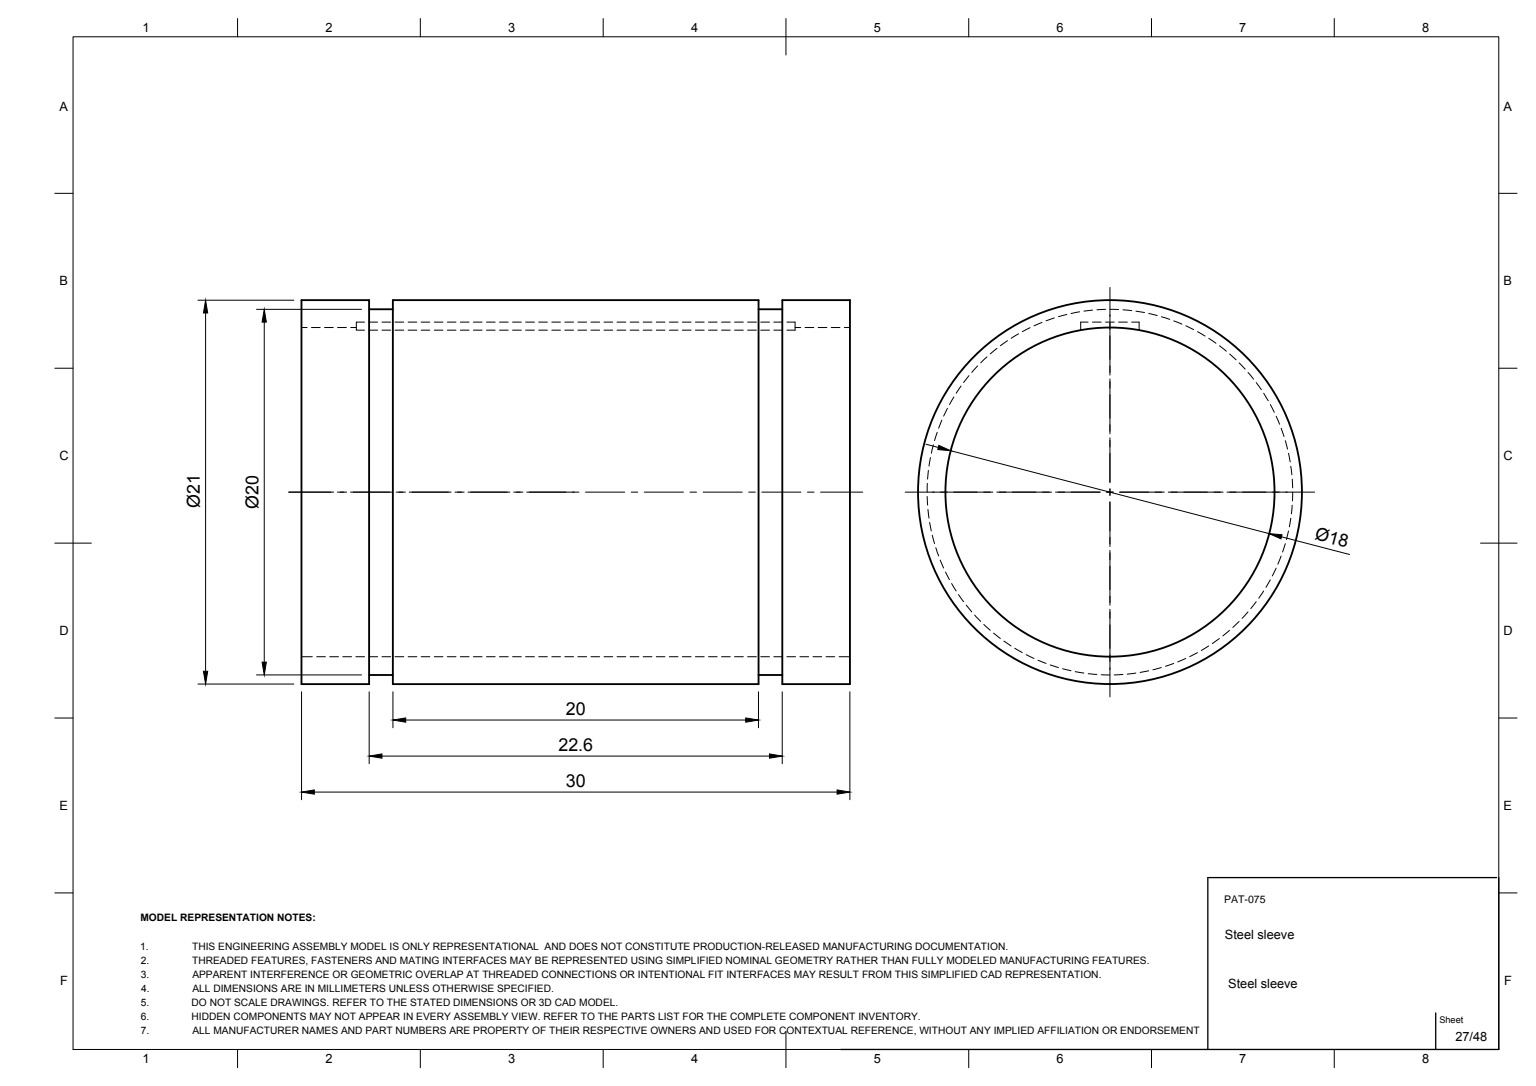
ISO-10303-21;
HEADER;
/* Generated by software containing ST-Developer
 * from STEP Tools, Inc. (www.steptools.com) 
 */

FILE_DESCRIPTION(
/* description */ ('Over-Centre Plunger Toggle Clamp on Slotted Fixture Frame'),
/* implementation_level */ '2;1');

FILE_NAME(
/* name */ 
'Steel sleeve.step',
/* time_stamp */ '2026-10-28T03:23:24-07:00',
/* author */ (''),
/* organization */ (''),
/* preprocessor_version */ 'ST-DEVELOPER v20.2',
/* originating_system */ 'Autodesk Translation Framework v15.17.0.0',
/* authorisation */ '');

FILE_SCHEMA (('AUTOMOTIVE_DESIGN { 1 0 10303 214 3 1 1 }'));
ENDSEC;

DATA;
#10=MECHANICAL_DESIGN_GEOMETRIC_PRESENTATION_REPRESENTATION('',(#542),#15212);
#450=SHAPE_REPRESENTATION_RELATIONSHIP('SRR','None',#15426,#492);
#492=ADVANCED_BREP_SHAPE_REPRESENTATION('',(#592),#15188);
#542=STYLED_ITEM('',(#15733),#592);
#592=MANIFOLD_SOLID_BREP('Body1',#8275);
#729=FACE_BOUND('',#1979,.T.);
#730=FACE_BOUND('',#1982,.T.);
#731=FACE_BOUND('',#1985,.T.);
#732=FACE_BOUND('',#1988,.T.);
#733=FACE_BOUND('',#1991,.T.);
#734=FACE_BOUND('',#1994,.T.);
#735=FACE_BOUND('',#1996,.T.);
#955=PLANE('',#9300);
#956=PLANE('',#9302);
#957=PLANE('',#9303);
#958=PLANE('',#9305);
#959=PLANE('',#9306);
#960=PLANE('',#9307);
#961=PLANE('',#9312);
#962=PLANE('',#9316);
#963=PLANE('',#9320);
#964=PLANE('',#9324);
#965=PLANE('',#9328);
#1369=FACE_OUTER_BOUND('',#1973,.T.);
#1370=FACE_OUTER_BOUND('',#1974,.T.);
#1371=FACE_OUTER_BOUND('',#1975,.T.);
#1372=FACE_OUTER_BOUND('',#1976,.T.);
#1373=FACE_OUTER_BOUND('',#1977,.T.);
#1374=FACE_OUTER_BOUND('',#1978,.T.);
#1375=FACE_OUTER_BOUND('',#1980,.T.);
#1376=FACE_OUTER_BOUND('',#1981,.T.);
#1377=FACE_OUTER_BOUND('',#1983,.T.);
#1378=FACE_OUTER_BOUND('',#1984,.T.);
#1379=FACE_OUTER_BOUND('',#1986,.T.);
#1380=FACE_OUTER_BOUND('',#1987,.T.);
#1381=FACE_OUTER_BOUND('',#1989,.T.);
#1382=FACE_OUTER_BOUND('',#1990,.T.);
#1383=FACE_OUTER_BOUND('',#1992,.T.);
#1384=FACE_OUTER_BOUND('',#1993,.T.);
#1385=FACE_OUTER_BOUND('',#1995,.T.);
#1973=EDGE_LOOP('',(#6841,#6842,#6843,#6844));
#1974=EDGE_LOOP('',(#6845,#6846,#6847,#6848));
#1975=EDGE_LOOP('',(#6849,#6850,#6851,#6852));
#1976=EDGE_LOOP('',(#6853,#6854,#6855,#6856));
#1977=EDGE_LOOP('',(#6857,#6858,#6859,#6860));
#1978=EDGE_LOOP('',(#6861));
#1979=EDGE_LOOP('',(#6862));
#1980=EDGE_LOOP('',(#6863,#6864,#6865,#6866));
#1981=EDGE_LOOP('',(#6867));
#1982=EDGE_LOOP('',(#6868));
#1983=EDGE_LOOP('',(#6869,#6870,#6871,#6872));
#1984=EDGE_LOOP('',(#6873));
#1985=EDGE_LOOP('',(#6874));
#1986=EDGE_LOOP('',(#6875,#6876,#6877,#6878));
#1987=EDGE_LOOP('',(#6879));
#1988=EDGE_LOOP('',(#6880));
#1989=EDGE_LOOP('',(#6881,#6882,#6883,#6884));
#1990=EDGE_LOOP('',(#6885));
#1991=EDGE_LOOP('',(#6886));
#1992=EDGE_LOOP('',(#6887,#6888,#6889,#6890));
#1993=EDGE_LOOP('',(#6891));
#1994=EDGE_LOOP('',(#6892));
#1995=EDGE_LOOP('',(#6893,#6894,#6895,#6896));
#1996=EDGE_LOOP('',(#6897,#6898,#6899,#6900));
#2625=LINE('',#14090,#3255);
#2626=LINE('',#14092,#3256);
#2627=LINE('',#14093,#3257);
#2628=LINE('',#14096,#3258);
#2629=LINE('',#14098,#3259);
#2630=LINE('',#14099,#3260);
#2631=LINE('',#14104,#3261);
#2632=LINE('',#14105,#3262);
#2633=LINE('',#14107,#3263);
#2634=LINE('',#14108,#3264);
#2635=LINE('',#14118,#3265);
#2636=LINE('',#14125,#3266);
#2637=LINE('',#14132,#3267);
#2638=LINE('',#14139,#3268);
#2639=LINE('',#14146,#3269);
#2640=LINE('',#14151,#3270);
#3255=VECTOR('',#11226,1.);
#3256=VECTOR('',#11227,1.);
#3257=VECTOR('',#11228,1.);
#3258=VECTOR('',#11231,1.);
#3259=VECTOR('',#11232,1.);
#3260=VECTOR('',#11233,1.);
#3261=VECTOR('',#11238,1.);
#3262=VECTOR('',#11239,1.);
#3263=VECTOR('',#11242,1.);
#3264=VECTOR('',#11243,1.);
#3265=VECTOR('',#11256,1.05);
#3266=VECTOR('',#11265,1.);
#3267=VECTOR('',#11274,1.05);
#3268=VECTOR('',#11283,1.);
#3269=VECTOR('',#11292,1.05);
#3270=VECTOR('',#11299,0.9);
#3713=CIRCLE('',#9301,0.9);
#3714=CIRCLE('',#9304,0.9);
#3715=CIRCLE('',#9308,1.05);
#3716=CIRCLE('',#9309,0.9);
#3717=CIRCLE('',#9311,1.05);
#3718=CIRCLE('',#9313,1.);
#3719=CIRCLE('',#9315,1.);
#3720=CIRCLE('',#9317,1.05);
#3721=CIRCLE('',#9319,1.05);
#3722=CIRCLE('',#9321,1.);
#3723=CIRCLE('',#9323,1.);
#3724=CIRCLE('',#9325,1.05);
#3725=CIRCLE('',#9327,1.05);
#3726=CIRCLE('',#9329,0.9);
#4291=VERTEX_POINT('',#14086);
#4292=VERTEX_POINT('',#14087);
#4293=VERTEX_POINT('',#14089);
#4294=VERTEX_POINT('',#14091);
#4295=VERTEX_POINT('',#14095);
#4296=VERTEX_POINT('',#14097);
#4297=VERTEX_POINT('',#14101);
#4298=VERTEX_POINT('',#14103);
#4299=VERTEX_POINT('',#14111);
#4300=VERTEX_POINT('',#14113);
#4301=VERTEX_POINT('',#14116);
#4302=VERTEX_POINT('',#14120);
#4303=VERTEX_POINT('',#14123);
#4304=VERTEX_POINT('',#14127);
#4305=VERTEX_POINT('',#14130);
#4306=VERTEX_POINT('',#14134);
#4307=VERTEX_POINT('',#14137);
#4308=VERTEX_POINT('',#14141);
#4309=VERTEX_POINT('',#14144);
#4310=VERTEX_POINT('',#14148);
#5181=EDGE_CURVE('',#4291,#4292,#3713,.T.);
#5182=EDGE_CURVE('',#4293,#4291,#2625,.T.);
#5183=EDGE_CURVE('',#4294,#4293,#2626,.T.);
#5184=EDGE_CURVE('',#4292,#4294,#2627,.T.);
#5185=EDGE_CURVE('',#4292,#4295,#2628,.T.);
#5186=EDGE_CURVE('',#4296,#4294,#2629,.T.);
#5187=EDGE_CURVE('',#4296,#4295,#2630,.T.);
#5188=EDGE_CURVE('',#4295,#4297,#3714,.T.);
#5189=EDGE_CURVE('',#4298,#4296,#2631,.T.);
#5190=EDGE_CURVE('',#4297,#4298,#2632,.T.);
#5191=EDGE_CURVE('',#4297,#4291,#2633,.T.);
#5192=EDGE_CURVE('',#4298,#4293,#2634,.T.);
#5193=EDGE_CURVE('',#4299,#4299,#3715,.T.);
#5194=EDGE_CURVE('',#4300,#4300,#3716,.T.);
#5195=EDGE_CURVE('',#4301,#4301,#3717,.T.);
#5196=EDGE_CURVE('',#4301,#4299,#2635,.T.);
#5197=EDGE_CURVE('',#4302,#4302,#3718,.T.);
#5198=EDGE_CURVE('',#4303,#4303,#3719,.T.);
#5199=EDGE_CURVE('',#4303,#4302,#2636,.T.);
#5200=EDGE_CURVE('',#4304,#4304,#3720,.T.);
#5201=EDGE_CURVE('',#4305,#4305,#3721,.T.);
#5202=EDGE_CURVE('',#4305,#4304,#2637,.T.);
#5203=EDGE_CURVE('',#4306,#4306,#3722,.T.);
#5204=EDGE_CURVE('',#4307,#4307,#3723,.T.);
#5205=EDGE_CURVE('',#4307,#4306,#2638,.T.);
#5206=EDGE_CURVE('',#4308,#4308,#3724,.T.);
#5207=EDGE_CURVE('',#4309,#4309,#3725,.T.);
#5208=EDGE_CURVE('',#4309,#4308,#2639,.T.);
#5209=EDGE_CURVE('',#4310,#4310,#3726,.T.);
#5210=EDGE_CURVE('',#4310,#4300,#2640,.T.);
#6841=ORIENTED_EDGE('',*,*,#5181,.F.);
#6842=ORIENTED_EDGE('',*,*,#5182,.F.);
#6843=ORIENTED_EDGE('',*,*,#5183,.F.);
#6844=ORIENTED_EDGE('',*,*,#5184,.F.);
#6845=ORIENTED_EDGE('',*,*,#5185,.F.);
#6846=ORIENTED_EDGE('',*,*,#5184,.T.);
#6847=ORIENTED_EDGE('',*,*,#5186,.F.);
#6848=ORIENTED_EDGE('',*,*,#5187,.T.);
#6849=ORIENTED_EDGE('',*,*,#5188,.F.);
#6850=ORIENTED_EDGE('',*,*,#5187,.F.);
#6851=ORIENTED_EDGE('',*,*,#5189,.F.);
#6852=ORIENTED_EDGE('',*,*,#5190,.F.);
#6853=ORIENTED_EDGE('',*,*,#5191,.F.);
#6854=ORIENTED_EDGE('',*,*,#5190,.T.);
#6855=ORIENTED_EDGE('',*,*,#5192,.T.);
#6856=ORIENTED_EDGE('',*,*,#5182,.T.);
#6857=ORIENTED_EDGE('',*,*,#5192,.F.);
#6858=ORIENTED_EDGE('',*,*,#5189,.T.);
#6859=ORIENTED_EDGE('',*,*,#5186,.T.);
#6860=ORIENTED_EDGE('',*,*,#5183,.T.);
#6861=ORIENTED_EDGE('',*,*,#5193,.F.);
#6862=ORIENTED_EDGE('',*,*,#5194,.T.);
#6863=ORIENTED_EDGE('',*,*,#5195,.F.);
#6864=ORIENTED_EDGE('',*,*,#5196,.T.);
#6865=ORIENTED_EDGE('',*,*,#5193,.T.);
#6866=ORIENTED_EDGE('',*,*,#5196,.F.);
#6867=ORIENTED_EDGE('',*,*,#5195,.T.);
#6868=ORIENTED_EDGE('',*,*,#5197,.F.);
#6869=ORIENTED_EDGE('',*,*,#5198,.F.);
#6870=ORIENTED_EDGE('',*,*,#5199,.T.);
#6871=ORIENTED_EDGE('',*,*,#5197,.T.);
#6872=ORIENTED_EDGE('',*,*,#5199,.F.);
#6873=ORIENTED_EDGE('',*,*,#5200,.F.);
#6874=ORIENTED_EDGE('',*,*,#5198,.T.);
#6875=ORIENTED_EDGE('',*,*,#5201,.F.);
#6876=ORIENTED_EDGE('',*,*,#5202,.T.);
#6877=ORIENTED_EDGE('',*,*,#5200,.T.);
#6878=ORIENTED_EDGE('',*,*,#5202,.F.);
#6879=ORIENTED_EDGE('',*,*,#5201,.T.);
#6880=ORIENTED_EDGE('',*,*,#5203,.F.);
#6881=ORIENTED_EDGE('',*,*,#5204,.F.);
#6882=ORIENTED_EDGE('',*,*,#5205,.T.);
#6883=ORIENTED_EDGE('',*,*,#5203,.T.);
#6884=ORIENTED_EDGE('',*,*,#5205,.F.);
#6885=ORIENTED_EDGE('',*,*,#5206,.F.);
#6886=ORIENTED_EDGE('',*,*,#5204,.T.);
#6887=ORIENTED_EDGE('',*,*,#5207,.F.);
#6888=ORIENTED_EDGE('',*,*,#5208,.T.);
#6889=ORIENTED_EDGE('',*,*,#5206,.T.);
#6890=ORIENTED_EDGE('',*,*,#5208,.F.);
#6891=ORIENTED_EDGE('',*,*,#5207,.T.);
#6892=ORIENTED_EDGE('',*,*,#5209,.F.);
#6893=ORIENTED_EDGE('',*,*,#5209,.T.);
#6894=ORIENTED_EDGE('',*,*,#5210,.T.);
#6895=ORIENTED_EDGE('',*,*,#5194,.F.);
#6896=ORIENTED_EDGE('',*,*,#5210,.F.);
#6897=ORIENTED_EDGE('',*,*,#5188,.T.);
#6898=ORIENTED_EDGE('',*,*,#5191,.T.);
#6899=ORIENTED_EDGE('',*,*,#5181,.T.);
#6900=ORIENTED_EDGE('',*,*,#5185,.T.);
#7701=CYLINDRICAL_SURFACE('',#9310,1.05);
#7702=CYLINDRICAL_SURFACE('',#9314,1.);
#7703=CYLINDRICAL_SURFACE('',#9318,1.05);
#7704=CYLINDRICAL_SURFACE('',#9322,1.);
#7705=CYLINDRICAL_SURFACE('',#9326,1.05);
#7706=CYLINDRICAL_SURFACE('',#9330,0.9);
#8041=ADVANCED_FACE('',(#1369),#955,.F.);
#8042=ADVANCED_FACE('',(#1370),#956,.F.);
#8043=ADVANCED_FACE('',(#1371),#957,.F.);
#8044=ADVANCED_FACE('',(#1372),#958,.F.);
#8045=ADVANCED_FACE('',(#1373),#959,.F.);
#8046=ADVANCED_FACE('',(#1374,#729),#960,.T.);
#8047=ADVANCED_FACE('',(#1375),#7701,.T.);
#8048=ADVANCED_FACE('',(#1376,#730),#961,.T.);
#8049=ADVANCED_FACE('',(#1377),#7702,.T.);
#8050=ADVANCED_FACE('',(#1378,#731),#962,.T.);
#8051=ADVANCED_FACE('',(#1379),#7703,.T.);
#8052=ADVANCED_FACE('',(#1380,#732),#963,.T.);
#8053=ADVANCED_FACE('',(#1381),#7704,.T.);
#8054=ADVANCED_FACE('',(#1382,#733),#964,.T.);
#8055=ADVANCED_FACE('',(#1383),#7705,.T.);
#8056=ADVANCED_FACE('',(#1384,#734),#965,.T.);
#8057=ADVANCED_FACE('',(#1385,#735),#7706,.F.);
#8275=CLOSED_SHELL('',(#8041,#8042,#8043,#8044,#8045,#8046,#8047,#8048,
#8049,#8050,#8051,#8052,#8053,#8054,#8055,#8056,#8057));
#9299=AXIS2_PLACEMENT_3D('',#14084,#11220,#11221);
#9300=AXIS2_PLACEMENT_3D('',#14085,#11222,#11223);
#9301=AXIS2_PLACEMENT_3D('',#14088,#11224,#11225);
#9302=AXIS2_PLACEMENT_3D('',#14094,#11229,#11230);
#9303=AXIS2_PLACEMENT_3D('',#14100,#11234,#11235);
#9304=AXIS2_PLACEMENT_3D('',#14102,#11236,#11237);
#9305=AXIS2_PLACEMENT_3D('',#14106,#11240,#11241);
#9306=AXIS2_PLACEMENT_3D('',#14109,#11244,#11245);
#9307=AXIS2_PLACEMENT_3D('',#14110,#11246,#11247);
#9308=AXIS2_PLACEMENT_3D('',#14112,#11248,#11249);
#9309=AXIS2_PLACEMENT_3D('',#14114,#11250,#11251);
#9310=AXIS2_PLACEMENT_3D('',#14115,#11252,#11253);
#9311=AXIS2_PLACEMENT_3D('',#14117,#11254,#11255);
#9312=AXIS2_PLACEMENT_3D('',#14119,#11257,#11258);
#9313=AXIS2_PLACEMENT_3D('',#14121,#11259,#11260);
#9314=AXIS2_PLACEMENT_3D('',#14122,#11261,#11262);
#9315=AXIS2_PLACEMENT_3D('',#14124,#11263,#11264);
#9316=AXIS2_PLACEMENT_3D('',#14126,#11266,#11267);
#9317=AXIS2_PLACEMENT_3D('',#14128,#11268,#11269);
#9318=AXIS2_PLACEMENT_3D('',#14129,#11270,#11271);
#9319=AXIS2_PLACEMENT_3D('',#14131,#11272,#11273);
#9320=AXIS2_PLACEMENT_3D('',#14133,#11275,#11276);
#9321=AXIS2_PLACEMENT_3D('',#14135,#11277,#11278);
#9322=AXIS2_PLACEMENT_3D('',#14136,#11279,#11280);
#9323=AXIS2_PLACEMENT_3D('',#14138,#11281,#11282);
#9324=AXIS2_PLACEMENT_3D('',#14140,#11284,#11285);
#9325=AXIS2_PLACEMENT_3D('',#14142,#11286,#11287);
#9326=AXIS2_PLACEMENT_3D('',#14143,#11288,#11289);
#9327=AXIS2_PLACEMENT_3D('',#14145,#11290,#11291);
#9328=AXIS2_PLACEMENT_3D('',#14147,#11293,#11294);
#9329=AXIS2_PLACEMENT_3D('',#14149,#11295,#11296);
#9330=AXIS2_PLACEMENT_3D('',#14150,#11297,#11298);
#11220=DIRECTION('axis',(0.,0.,1.));
#11221=DIRECTION('refdir',(1.,0.,0.));
#11222=DIRECTION('center_axis',(0.,1.,0.));
#11223=DIRECTION('ref_axis',(0.,0.,1.));
#11224=DIRECTION('center_axis',(0.,-1.,0.));
#11225=DIRECTION('ref_axis',(1.,0.,0.));
#11226=DIRECTION('',(-1.,0.,0.));
#11227=DIRECTION('',(0.,0.,-1.));
#11228=DIRECTION('',(1.,0.,0.));
#11229=DIRECTION('center_axis',(0.,0.,1.));
#11230=DIRECTION('ref_axis',(1.,0.,0.));
#11231=DIRECTION('',(0.,-1.,0.));
#11232=DIRECTION('',(0.,1.,0.));
#11233=DIRECTION('',(-1.,0.,0.));
#11234=DIRECTION('center_axis',(0.,-1.,0.));
#11235=DIRECTION('ref_axis',(0.,0.,-1.));
#11236=DIRECTION('center_axis',(0.,1.,0.));
#11237=DIRECTION('ref_axis',(1.,0.,0.));
#11238=DIRECTION('',(0.,0.,1.));
#11239=DIRECTION('',(1.,0.,0.));
#11240=DIRECTION('center_axis',(0.,0.,-1.));
#11241=DIRECTION('ref_axis',(-1.,0.,0.));
#11242=DIRECTION('',(0.,1.,0.));
#11243=DIRECTION('',(0.,1.,0.));
#11244=DIRECTION('center_axis',(1.,0.,0.));
#11245=DIRECTION('ref_axis',(0.,0.,-1.));
#11246=DIRECTION('center_axis',(0.,1.,0.));
#11247=DIRECTION('ref_axis',(0.,0.,1.));
#11248=DIRECTION('center_axis',(0.,-1.,0.));
#11249=DIRECTION('ref_axis',(1.,0.,0.));
#11250=DIRECTION('center_axis',(0.,-1.,0.));
#11251=DIRECTION('ref_axis',(1.,0.,0.));
#11252=DIRECTION('center_axis',(0.,-1.,0.));
#11253=DIRECTION('ref_axis',(1.,0.,0.));
#11254=DIRECTION('center_axis',(0.,-1.,0.));
#11255=DIRECTION('ref_axis',(1.,0.,0.));
#11256=DIRECTION('',(0.,1.,0.));
#11257=DIRECTION('center_axis',(0.,-1.,0.));
#11258=DIRECTION('ref_axis',(0.,0.,-1.));
#11259=DIRECTION('center_axis',(0.,-1.,0.));
#11260=DIRECTION('ref_axis',(1.,0.,0.));
#11261=DIRECTION('center_axis',(0.,-1.,0.));
#11262=DIRECTION('ref_axis',(1.,0.,0.));
#11263=DIRECTION('center_axis',(0.,-1.,0.));
#11264=DIRECTION('ref_axis',(1.,0.,0.));
#11265=DIRECTION('',(0.,1.,0.));
#11266=DIRECTION('center_axis',(0.,1.,0.));
#11267=DIRECTION('ref_axis',(0.,0.,1.));
#11268=DIRECTION('center_axis',(0.,-1.,0.));
#11269=DIRECTION('ref_axis',(1.,0.,0.));
#11270=DIRECTION('center_axis',(0.,-1.,0.));
#11271=DIRECTION('ref_axis',(1.,0.,0.));
#11272=DIRECTION('center_axis',(0.,-1.,0.));
#11273=DIRECTION('ref_axis',(1.,0.,0.));
#11274=DIRECTION('',(0.,1.,0.));
#11275=DIRECTION('center_axis',(0.,-1.,0.));
#11276=DIRECTION('ref_axis',(0.,0.,-1.));
#11277=DIRECTION('center_axis',(0.,-1.,0.));
#11278=DIRECTION('ref_axis',(1.,0.,0.));
#11279=DIRECTION('center_axis',(0.,-1.,0.));
#11280=DIRECTION('ref_axis',(1.,0.,0.));
#11281=DIRECTION('center_axis',(0.,-1.,0.));
#11282=DIRECTION('ref_axis',(1.,0.,0.));
#11283=DIRECTION('',(0.,1.,0.));
#11284=DIRECTION('center_axis',(0.,1.,0.));
#11285=DIRECTION('ref_axis',(0.,0.,1.));
#11286=DIRECTION('center_axis',(0.,-1.,0.));
#11287=DIRECTION('ref_axis',(1.,0.,0.));
#11288=DIRECTION('center_axis',(0.,-1.,0.));
#11289=DIRECTION('ref_axis',(1.,0.,0.));
#11290=DIRECTION('center_axis',(0.,-1.,0.));
#11291=DIRECTION('ref_axis',(1.,0.,0.));
#11292=DIRECTION('',(0.,1.,0.));
#11293=DIRECTION('center_axis',(0.,-1.,0.));
#11294=DIRECTION('ref_axis',(0.,0.,-1.));
#11295=DIRECTION('center_axis',(0.,-1.,0.));
#11296=DIRECTION('ref_axis',(1.,0.,0.));
#11297=DIRECTION('center_axis',(0.,-1.,0.));
#11298=DIRECTION('ref_axis',(1.,0.,0.));
#11299=DIRECTION('',(0.,1.,0.));
#14084=CARTESIAN_POINT('',(0.,0.,0.));
#14085=CARTESIAN_POINT('Origin',(0.75,1.2,0.));
#14086=CARTESIAN_POINT('',(0.885663593019381,1.2,-0.16));
#14087=CARTESIAN_POINT('',(0.885663593019381,1.2,0.16));
#14088=CARTESIAN_POINT('Origin',(0.,1.2,0.));
#14089=CARTESIAN_POINT('',(0.93,1.2,-0.16));
#14090=CARTESIAN_POINT('',(0.93,1.2,-0.16));
#14091=CARTESIAN_POINT('',(0.93,1.2,0.16));
#14092=CARTESIAN_POINT('',(0.93,1.2,0.16));
#14093=CARTESIAN_POINT('',(0.57,1.2,0.16));
#14094=CARTESIAN_POINT('Origin',(0.57,0.,0.16));
#14095=CARTESIAN_POINT('',(0.885663593019381,-1.2,0.16));
#14096=CARTESIAN_POINT('',(0.885663593019381,0.,0.16));
#14097=CARTESIAN_POINT('',(0.93,-1.2,0.16));
#14098=CARTESIAN_POINT('',(0.93,0.,0.16));
#14099=CARTESIAN_POINT('',(0.57,-1.2,0.16));
#14100=CARTESIAN_POINT('Origin',(0.75,-1.2,0.));
#14101=CARTESIAN_POINT('',(0.885663593019381,-1.2,-0.16));
#14102=CARTESIAN_POINT('Origin',(0.,-1.2,0.));
#14103=CARTESIAN_POINT('',(0.93,-1.2,-0.16));
#14104=CARTESIAN_POINT('',(0.93,-1.2,0.16));
#14105=CARTESIAN_POINT('',(0.93,-1.2,-0.16));
#14106=CARTESIAN_POINT('Origin',(0.93,0.,-0.16));
#14107=CARTESIAN_POINT('',(0.885663593019381,0.,-0.16));
#14108=CARTESIAN_POINT('',(0.93,0.,-0.16));
#14109=CARTESIAN_POINT('Origin',(0.93,0.,0.16));
#14110=CARTESIAN_POINT('Origin',(1.05,1.5,0.));
#14111=CARTESIAN_POINT('',(-1.05,1.5,-1.28587913910472E-16));
#14112=CARTESIAN_POINT('Origin',(0.,1.5,0.));
#14113=CARTESIAN_POINT('',(-0.9,1.5,-1.10218211923262E-16));
#14114=CARTESIAN_POINT('Origin',(0.,1.5,0.));
#14115=CARTESIAN_POINT('Origin',(0.,1.315,0.));
#14116=CARTESIAN_POINT('',(-1.05,1.13,-1.28587913910472E-16));
#14117=CARTESIAN_POINT('Origin',(0.,1.13,0.));
#14118=CARTESIAN_POINT('',(-1.05,1.315,-1.28587913910472E-16));
#14119=CARTESIAN_POINT('Origin',(1.,1.13,0.));
#14120=CARTESIAN_POINT('',(-1.,1.13,-1.22464679914735E-16));
#14121=CARTESIAN_POINT('Origin',(0.,1.13,0.));
#14122=CARTESIAN_POINT('Origin',(0.,1.065,0.));
#14123=CARTESIAN_POINT('',(-1.,1.,-1.22464679914735E-16));
#14124=CARTESIAN_POINT('Origin',(0.,1.,0.));
#14125=CARTESIAN_POINT('',(-1.,1.065,-1.22464679914735E-16));
#14126=CARTESIAN_POINT('Origin',(1.05,1.,0.));
#14127=CARTESIAN_POINT('',(-1.05,1.,-1.28587913910472E-16));
#14128=CARTESIAN_POINT('Origin',(0.,1.,0.));
#14129=CARTESIAN_POINT('Origin',(0.,0.,0.));
#14130=CARTESIAN_POINT('',(-1.05,-1.,-1.28587913910472E-16));
#14131=CARTESIAN_POINT('Origin',(0.,-1.,0.));
#14132=CARTESIAN_POINT('',(-1.05,0.,-1.28587913910472E-16));
#14133=CARTESIAN_POINT('Origin',(1.,-1.,0.));
#14134=CARTESIAN_POINT('',(-1.,-1.,-1.22464679914735E-16));
#14135=CARTESIAN_POINT('Origin',(0.,-1.,0.));
#14136=CARTESIAN_POINT('Origin',(0.,-1.065,0.));
#14137=CARTESIAN_POINT('',(-1.,-1.13,-1.22464679914735E-16));
#14138=CARTESIAN_POINT('Origin',(0.,-1.13,0.));
#14139=CARTESIAN_POINT('',(-1.,-1.065,-1.22464679914735E-16));
#14140=CARTESIAN_POINT('Origin',(1.05,-1.13,0.));
#14141=CARTESIAN_POINT('',(-1.05,-1.13,-1.28587913910472E-16));
#14142=CARTESIAN_POINT('Origin',(0.,-1.13,0.));
#14143=CARTESIAN_POINT('Origin',(0.,-1.315,0.));
#14144=CARTESIAN_POINT('',(-1.05,-1.5,-1.28587913910472E-16));
#14145=CARTESIAN_POINT('Origin',(0.,-1.5,0.));
#14146=CARTESIAN_POINT('',(-1.05,-1.315,-1.28587913910472E-16));
#14147=CARTESIAN_POINT('Origin',(0.9,-1.5,0.));
#14148=CARTESIAN_POINT('',(-0.9,-1.5,-1.10218211923262E-16));
#14149=CARTESIAN_POINT('Origin',(0.,-1.5,0.));
#14150=CARTESIAN_POINT('Origin',(0.,0.,0.));
#14151=CARTESIAN_POINT('',(-0.9,0.,-1.10218211923262E-16));
#15138=UNCERTAINTY_MEASURE_WITH_UNIT(LENGTH_MEASURE(0.001),#15213,
'DISTANCE_ACCURACY_VALUE',
'Maximum model space distance between geometric entities at asserted c
onnectivities');
#15162=UNCERTAINTY_MEASURE_WITH_UNIT(LENGTH_MEASURE(0.001),#15213,
'DISTANCE_ACCURACY_VALUE',
'Maximum model space distance between geometric entities at asserted c
onnectivities');
#15188=(
GEOMETRIC_REPRESENTATION_CONTEXT(3)
GLOBAL_UNCERTAINTY_ASSIGNED_CONTEXT((#15138))
GLOBAL_UNIT_ASSIGNED_CONTEXT((#15213,#15215,#15216))
REPRESENTATION_CONTEXT('','3D')
);
#15212=(
GEOMETRIC_REPRESENTATION_CONTEXT(3)
GLOBAL_UNCERTAINTY_ASSIGNED_CONTEXT((#15162))
GLOBAL_UNIT_ASSIGNED_CONTEXT((#15213,#15215,#15216))
REPRESENTATION_CONTEXT('','3D')
);
#15213=(
LENGTH_UNIT()
NAMED_UNIT(*)
SI_UNIT(.CENTI.,.METRE.)
);
#15215=(
NAMED_UNIT(*)
PLANE_ANGLE_UNIT()
SI_UNIT($,.RADIAN.)
);
#15216=(
NAMED_UNIT(*)
SI_UNIT($,.STERADIAN.)
SOLID_ANGLE_UNIT()
);
#15242=SHAPE_DEFINITION_REPRESENTATION(#15296,#15426);
#15296=PRODUCT_DEFINITION_SHAPE('',$,#15476);
#15426=SHAPE_REPRESENTATION('',(#9299),#15188);
#15450=PRODUCT_DEFINITION_CONTEXT('part definition',#15599,'design');
#15476=PRODUCT_DEFINITION('Steel sleeve','Steel sleeve',#15525,#15450);
#15525=PRODUCT_DEFINITION_FORMATION('',$,#15626);
#15599=APPLICATION_CONTEXT(
'Core Data for Automotive Mechanical Design Process');
#15600=PRODUCT_CONTEXT('part definition',#15599,'mechanical');
#15626=PRODUCT('Steel sleeve','Steel sleeve','Steel sleeve',(#15600));
#15727=COLOUR_RGB('Off White',0.89,0.88,0.83);
#15728=FILL_AREA_STYLE_COLOUR('',#15727);
#15729=FILL_AREA_STYLE('',(#15728));
#15730=SURFACE_STYLE_FILL_AREA(#15729);
#15731=SURFACE_SIDE_STYLE('',(#15730));
#15732=SURFACE_STYLE_USAGE(.BOTH.,#15731);
#15733=PRESENTATION_STYLE_ASSIGNMENT((#15732));
ENDSEC;
END-ISO-10303-21;
